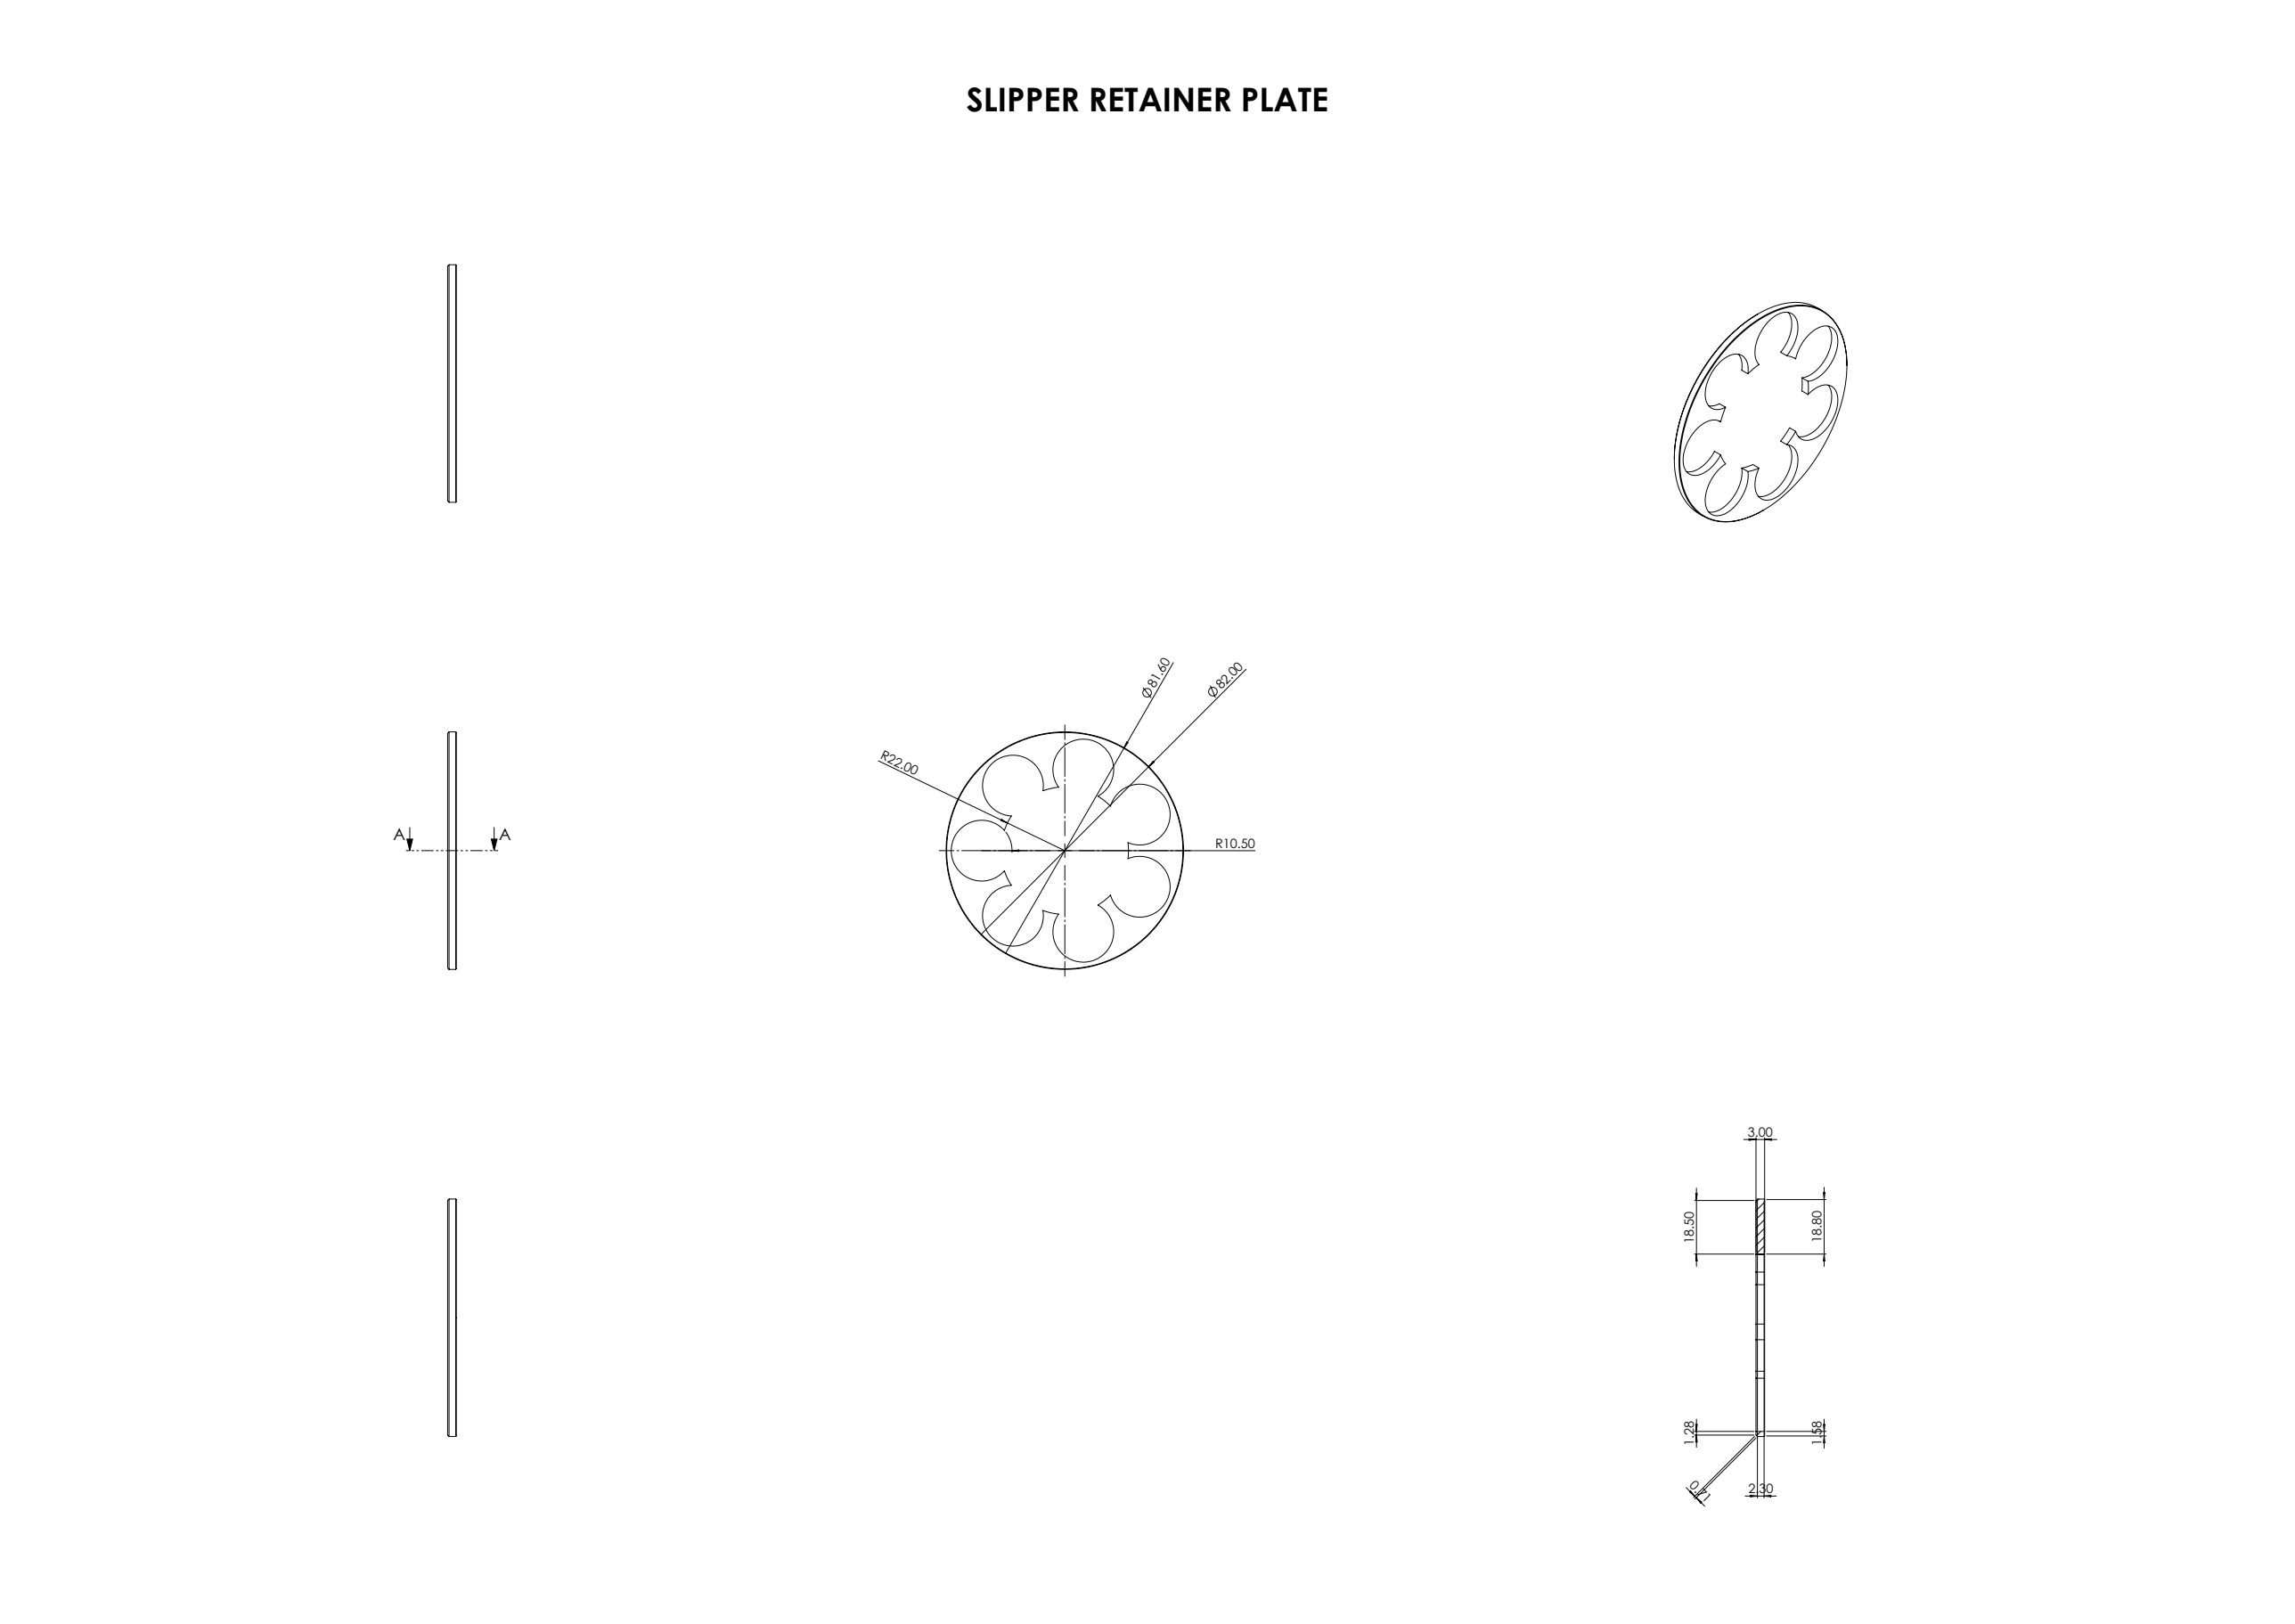
ISO-10303-21;
HEADER;
/* Generated by software containing ST-Developer
 * from STEP Tools, Inc. (www.steptools.com) 
 */

FILE_DESCRIPTION(
/* description */ (''),
/* implementation_level */ '2;1');

FILE_NAME(
/* name */ '07_Slipper_Retainer_Plate.step',
/* time_stamp */ '2026-10-26T07:49:00-07:00',
/* author */ (''),
/* organization */ (''),
/* preprocessor_version */ 'ST-DEVELOPER v20.2',
/* originating_system */ 'Autodesk Translation Framework v15.15.0.0',
/* authorisation */ '');

FILE_SCHEMA (('AUTOMOTIVE_DESIGN { 1 0 10303 214 3 1 1 }'));
ENDSEC;

DATA;
#10=MECHANICAL_DESIGN_GEOMETRIC_PRESENTATION_REPRESENTATION('',(#189),#38507);
#159=SHAPE_REPRESENTATION_RELATIONSHIP('SRR','None',#38587,#174);
#174=ADVANCED_BREP_SHAPE_REPRESENTATION('',(#204),#38504);
#189=STYLED_ITEM('',(#38713),#204);
#204=MANIFOLD_SOLID_BREP('Body1',#15083);
#515=FACE_BOUND('',#3178,.T.);
#516=FACE_BOUND('',#3194,.T.);
#809=PLANE('',#16309);
#810=PLANE('',#16352);
#1513=CYLINDRICAL_SURFACE('',#16324,41.);
#1514=CYLINDRICAL_SURFACE('',#16326,10.5);
#1515=CYLINDRICAL_SURFACE('',#16328,22.);
#1516=CYLINDRICAL_SURFACE('',#16330,10.5);
#1517=CYLINDRICAL_SURFACE('',#16332,22.);
#1518=CYLINDRICAL_SURFACE('',#16334,10.5);
#1519=CYLINDRICAL_SURFACE('',#16336,22.);
#1520=CYLINDRICAL_SURFACE('',#16338,10.5);
#1521=CYLINDRICAL_SURFACE('',#16340,22.);
#1522=CYLINDRICAL_SURFACE('',#16342,10.5);
#1523=CYLINDRICAL_SURFACE('',#16344,22.);
#1524=CYLINDRICAL_SURFACE('',#16346,10.5);
#1525=CYLINDRICAL_SURFACE('',#16348,22.);
#1526=CYLINDRICAL_SURFACE('',#16350,10.5);
#1527=CYLINDRICAL_SURFACE('',#16355,22.);
#2191=FACE_OUTER_BOUND('',#3176,.T.);
#2192=FACE_OUTER_BOUND('',#3177,.T.);
#2193=FACE_OUTER_BOUND('',#3179,.T.);
#2194=FACE_OUTER_BOUND('',#3180,.T.);
#2195=FACE_OUTER_BOUND('',#3181,.T.);
#2196=FACE_OUTER_BOUND('',#3182,.T.);
#2197=FACE_OUTER_BOUND('',#3183,.T.);
#2198=FACE_OUTER_BOUND('',#3184,.T.);
#2199=FACE_OUTER_BOUND('',#3185,.T.);
#2200=FACE_OUTER_BOUND('',#3186,.T.);
#2201=FACE_OUTER_BOUND('',#3187,.T.);
#2202=FACE_OUTER_BOUND('',#3188,.T.);
#2203=FACE_OUTER_BOUND('',#3189,.T.);
#2204=FACE_OUTER_BOUND('',#3190,.T.);
#2205=FACE_OUTER_BOUND('',#3191,.T.);
#2206=FACE_OUTER_BOUND('',#3192,.T.);
#2207=FACE_OUTER_BOUND('',#3193,.T.);
#2208=FACE_OUTER_BOUND('',#3195,.T.);
#2209=FACE_OUTER_BOUND('',#3196,.T.);
#3176=EDGE_LOOP('',(#12565,#12566,#12567,#12568,#12569));
#3177=EDGE_LOOP('',(#12570));
#3178=EDGE_LOOP('',(#12571,#12572,#12573,#12574,#12575,#12576,#12577,#12578,
#12579,#12580,#12581,#12582,#12583,#12584));
#3179=EDGE_LOOP('',(#12585,#12586,#12587,#12588,#12589));
#3180=EDGE_LOOP('',(#12590,#12591,#12592,#12593));
#3181=EDGE_LOOP('',(#12594,#12595,#12596,#12597));
#3182=EDGE_LOOP('',(#12598,#12599,#12600,#12601));
#3183=EDGE_LOOP('',(#12602,#12603,#12604,#12605));
#3184=EDGE_LOOP('',(#12606,#12607,#12608,#12609));
#3185=EDGE_LOOP('',(#12610,#12611,#12612,#12613));
#3186=EDGE_LOOP('',(#12614,#12615,#12616,#12617));
#3187=EDGE_LOOP('',(#12618,#12619,#12620,#12621));
#3188=EDGE_LOOP('',(#12622,#12623,#12624,#12625));
#3189=EDGE_LOOP('',(#12626,#12627,#12628,#12629));
#3190=EDGE_LOOP('',(#12630,#12631,#12632,#12633));
#3191=EDGE_LOOP('',(#12634,#12635,#12636,#12637));
#3192=EDGE_LOOP('',(#12638,#12639,#12640,#12641));
#3193=EDGE_LOOP('',(#12642));
#3194=EDGE_LOOP('',(#12643,#12644,#12645,#12646,#12647,#12648,#12649,#12650,
#12651,#12652,#12653,#12654,#12655,#12656));
#3195=EDGE_LOOP('',(#12657,#12658,#12659,#12660));
#3196=EDGE_LOOP('',(#12661,#12662,#12663,#12664));
#4141=LINE('',#27131,#5210);
#4142=LINE('',#27166,#5211);
#4143=LINE('',#27172,#5212);
#4144=LINE('',#27173,#5213);
#4145=LINE('',#27177,#5214);
#4146=LINE('',#27181,#5215);
#4147=LINE('',#27185,#5216);
#4148=LINE('',#27189,#5217);
#4149=LINE('',#27193,#5218);
#4150=LINE('',#27197,#5219);
#4151=LINE('',#27201,#5220);
#4152=LINE('',#27205,#5221);
#4153=LINE('',#27209,#5222);
#4154=LINE('',#27213,#5223);
#4155=LINE('',#27217,#5224);
#4156=LINE('',#27221,#5225);
#4157=LINE('',#27228,#5226);
#5210=VECTOR('',#19494,40.9);
#5211=VECTOR('',#19531,41.);
#5212=VECTOR('',#19538,10.);
#5213=VECTOR('',#19539,10.);
#5214=VECTOR('',#19544,10.);
#5215=VECTOR('',#19549,10.);
#5216=VECTOR('',#19554,10.);
#5217=VECTOR('',#19559,10.);
#5218=VECTOR('',#19564,10.);
#5219=VECTOR('',#19569,10.);
#5220=VECTOR('',#19574,10.);
#5221=VECTOR('',#19579,10.);
#5222=VECTOR('',#19584,10.);
#5223=VECTOR('',#19589,10.);
#5224=VECTOR('',#19594,10.);
#5225=VECTOR('',#19599,10.);
#5226=VECTOR('',#19610,40.75);
#6142=CIRCLE('',#16306,40.8);
#6143=CIRCLE('',#16307,41.);
#6144=CIRCLE('',#16308,41.);
#6145=CIRCLE('',#16310,10.5);
#6146=CIRCLE('',#16311,22.);
#6147=CIRCLE('',#16312,10.5);
#6148=CIRCLE('',#16313,22.);
#6149=CIRCLE('',#16314,10.5);
#6150=CIRCLE('',#16315,22.);
#6151=CIRCLE('',#16316,10.5);
#6152=CIRCLE('',#16317,22.);
#6153=CIRCLE('',#16318,10.5);
#6154=CIRCLE('',#16319,22.);
#6155=CIRCLE('',#16320,10.5);
#6156=CIRCLE('',#16321,22.);
#6157=CIRCLE('',#16322,10.5);
#6158=CIRCLE('',#16323,22.);
#6159=CIRCLE('',#16325,41.);
#6160=CIRCLE('',#16327,10.5);
#6161=CIRCLE('',#16329,22.);
#6162=CIRCLE('',#16331,10.5);
#6163=CIRCLE('',#16333,22.);
#6164=CIRCLE('',#16335,10.5);
#6165=CIRCLE('',#16337,22.);
#6166=CIRCLE('',#16339,10.5);
#6167=CIRCLE('',#16341,22.);
#6168=CIRCLE('',#16343,10.5);
#6169=CIRCLE('',#16345,22.);
#6170=CIRCLE('',#16347,10.5);
#6171=CIRCLE('',#16349,22.);
#6172=CIRCLE('',#16351,10.5);
#6173=CIRCLE('',#16353,40.5);
#6174=CIRCLE('',#16354,22.);
#7146=VERTEX_POINT('',#27128);
#7147=VERTEX_POINT('',#27130);
#7148=VERTEX_POINT('',#27132);
#7149=VERTEX_POINT('',#27136);
#7150=VERTEX_POINT('',#27137);
#7151=VERTEX_POINT('',#27139);
#7152=VERTEX_POINT('',#27141);
#7153=VERTEX_POINT('',#27143);
#7154=VERTEX_POINT('',#27145);
#7155=VERTEX_POINT('',#27147);
#7156=VERTEX_POINT('',#27149);
#7157=VERTEX_POINT('',#27151);
#7158=VERTEX_POINT('',#27153);
#7159=VERTEX_POINT('',#27155);
#7160=VERTEX_POINT('',#27157);
#7161=VERTEX_POINT('',#27159);
#7162=VERTEX_POINT('',#27161);
#7163=VERTEX_POINT('',#27165);
#7164=VERTEX_POINT('',#27169);
#7165=VERTEX_POINT('',#27170);
#7166=VERTEX_POINT('',#27175);
#7167=VERTEX_POINT('',#27179);
#7168=VERTEX_POINT('',#27183);
#7169=VERTEX_POINT('',#27187);
#7170=VERTEX_POINT('',#27191);
#7171=VERTEX_POINT('',#27195);
#7172=VERTEX_POINT('',#27199);
#7173=VERTEX_POINT('',#27203);
#7174=VERTEX_POINT('',#27207);
#7175=VERTEX_POINT('',#27211);
#7176=VERTEX_POINT('',#27215);
#7177=VERTEX_POINT('',#27219);
#7178=VERTEX_POINT('',#27223);
#9031=EDGE_CURVE('',#7146,#7146,#6142,.T.);
#9032=EDGE_CURVE('',#7146,#7147,#4141,.T.);
#9033=EDGE_CURVE('',#7147,#7148,#6143,.T.);
#9034=EDGE_CURVE('',#7148,#7147,#6144,.T.);
#9035=EDGE_CURVE('',#7149,#7150,#6145,.T.);
#9036=EDGE_CURVE('',#7151,#7150,#6146,.T.);
#9037=EDGE_CURVE('',#7151,#7152,#6147,.T.);
#9038=EDGE_CURVE('',#7153,#7152,#6148,.T.);
#9039=EDGE_CURVE('',#7153,#7154,#6149,.T.);
#9040=EDGE_CURVE('',#7155,#7154,#6150,.T.);
#9041=EDGE_CURVE('',#7155,#7156,#6151,.T.);
#9042=EDGE_CURVE('',#7157,#7156,#6152,.T.);
#9043=EDGE_CURVE('',#7157,#7158,#6153,.T.);
#9044=EDGE_CURVE('',#7159,#7158,#6154,.T.);
#9045=EDGE_CURVE('',#7159,#7160,#6155,.T.);
#9046=EDGE_CURVE('',#7161,#7160,#6156,.T.);
#9047=EDGE_CURVE('',#7161,#7162,#6157,.T.);
#9048=EDGE_CURVE('',#7149,#7162,#6158,.T.);
#9049=EDGE_CURVE('',#7148,#7163,#4142,.T.);
#9050=EDGE_CURVE('',#7163,#7163,#6159,.T.);
#9051=EDGE_CURVE('',#7164,#7165,#6160,.T.);
#9052=EDGE_CURVE('',#7150,#7164,#4143,.T.);
#9053=EDGE_CURVE('',#7165,#7149,#4144,.T.);
#9054=EDGE_CURVE('',#7166,#7164,#6161,.T.);
#9055=EDGE_CURVE('',#7166,#7151,#4145,.T.);
#9056=EDGE_CURVE('',#7167,#7166,#6162,.T.);
#9057=EDGE_CURVE('',#7152,#7167,#4146,.T.);
#9058=EDGE_CURVE('',#7168,#7167,#6163,.T.);
#9059=EDGE_CURVE('',#7168,#7153,#4147,.T.);
#9060=EDGE_CURVE('',#7169,#7168,#6164,.T.);
#9061=EDGE_CURVE('',#7154,#7169,#4148,.T.);
#9062=EDGE_CURVE('',#7170,#7169,#6165,.T.);
#9063=EDGE_CURVE('',#7170,#7155,#4149,.T.);
#9064=EDGE_CURVE('',#7171,#7170,#6166,.T.);
#9065=EDGE_CURVE('',#7156,#7171,#4150,.T.);
#9066=EDGE_CURVE('',#7172,#7171,#6167,.T.);
#9067=EDGE_CURVE('',#7172,#7157,#4151,.T.);
#9068=EDGE_CURVE('',#7173,#7172,#6168,.T.);
#9069=EDGE_CURVE('',#7158,#7173,#4152,.T.);
#9070=EDGE_CURVE('',#7174,#7173,#6169,.T.);
#9071=EDGE_CURVE('',#7174,#7159,#4153,.T.);
#9072=EDGE_CURVE('',#7175,#7174,#6170,.T.);
#9073=EDGE_CURVE('',#7160,#7175,#4154,.T.);
#9074=EDGE_CURVE('',#7176,#7175,#6171,.T.);
#9075=EDGE_CURVE('',#7176,#7161,#4155,.T.);
#9076=EDGE_CURVE('',#7177,#7176,#6172,.T.);
#9077=EDGE_CURVE('',#7162,#7177,#4156,.T.);
#9078=EDGE_CURVE('',#7178,#7178,#6173,.T.);
#9079=EDGE_CURVE('',#7165,#7177,#6174,.T.);
#9080=EDGE_CURVE('',#7163,#7178,#4157,.T.);
#12565=ORIENTED_EDGE('',*,*,#9031,.T.);
#12566=ORIENTED_EDGE('',*,*,#9032,.T.);
#12567=ORIENTED_EDGE('',*,*,#9033,.T.);
#12568=ORIENTED_EDGE('',*,*,#9034,.T.);
#12569=ORIENTED_EDGE('',*,*,#9032,.F.);
#12570=ORIENTED_EDGE('',*,*,#9031,.F.);
#12571=ORIENTED_EDGE('',*,*,#9035,.T.);
#12572=ORIENTED_EDGE('',*,*,#9036,.F.);
#12573=ORIENTED_EDGE('',*,*,#9037,.T.);
#12574=ORIENTED_EDGE('',*,*,#9038,.F.);
#12575=ORIENTED_EDGE('',*,*,#9039,.T.);
#12576=ORIENTED_EDGE('',*,*,#9040,.F.);
#12577=ORIENTED_EDGE('',*,*,#9041,.T.);
#12578=ORIENTED_EDGE('',*,*,#9042,.F.);
#12579=ORIENTED_EDGE('',*,*,#9043,.T.);
#12580=ORIENTED_EDGE('',*,*,#9044,.F.);
#12581=ORIENTED_EDGE('',*,*,#9045,.T.);
#12582=ORIENTED_EDGE('',*,*,#9046,.F.);
#12583=ORIENTED_EDGE('',*,*,#9047,.T.);
#12584=ORIENTED_EDGE('',*,*,#9048,.F.);
#12585=ORIENTED_EDGE('',*,*,#9033,.F.);
#12586=ORIENTED_EDGE('',*,*,#9034,.F.);
#12587=ORIENTED_EDGE('',*,*,#9049,.T.);
#12588=ORIENTED_EDGE('',*,*,#9050,.T.);
#12589=ORIENTED_EDGE('',*,*,#9049,.F.);
#12590=ORIENTED_EDGE('',*,*,#9051,.F.);
#12591=ORIENTED_EDGE('',*,*,#9052,.F.);
#12592=ORIENTED_EDGE('',*,*,#9035,.F.);
#12593=ORIENTED_EDGE('',*,*,#9053,.F.);
#12594=ORIENTED_EDGE('',*,*,#9052,.T.);
#12595=ORIENTED_EDGE('',*,*,#9054,.F.);
#12596=ORIENTED_EDGE('',*,*,#9055,.T.);
#12597=ORIENTED_EDGE('',*,*,#9036,.T.);
#12598=ORIENTED_EDGE('',*,*,#9056,.F.);
#12599=ORIENTED_EDGE('',*,*,#9057,.F.);
#12600=ORIENTED_EDGE('',*,*,#9037,.F.);
#12601=ORIENTED_EDGE('',*,*,#9055,.F.);
#12602=ORIENTED_EDGE('',*,*,#9057,.T.);
#12603=ORIENTED_EDGE('',*,*,#9058,.F.);
#12604=ORIENTED_EDGE('',*,*,#9059,.T.);
#12605=ORIENTED_EDGE('',*,*,#9038,.T.);
#12606=ORIENTED_EDGE('',*,*,#9060,.F.);
#12607=ORIENTED_EDGE('',*,*,#9061,.F.);
#12608=ORIENTED_EDGE('',*,*,#9039,.F.);
#12609=ORIENTED_EDGE('',*,*,#9059,.F.);
#12610=ORIENTED_EDGE('',*,*,#9061,.T.);
#12611=ORIENTED_EDGE('',*,*,#9062,.F.);
#12612=ORIENTED_EDGE('',*,*,#9063,.T.);
#12613=ORIENTED_EDGE('',*,*,#9040,.T.);
#12614=ORIENTED_EDGE('',*,*,#9064,.F.);
#12615=ORIENTED_EDGE('',*,*,#9065,.F.);
#12616=ORIENTED_EDGE('',*,*,#9041,.F.);
#12617=ORIENTED_EDGE('',*,*,#9063,.F.);
#12618=ORIENTED_EDGE('',*,*,#9065,.T.);
#12619=ORIENTED_EDGE('',*,*,#9066,.F.);
#12620=ORIENTED_EDGE('',*,*,#9067,.T.);
#12621=ORIENTED_EDGE('',*,*,#9042,.T.);
#12622=ORIENTED_EDGE('',*,*,#9068,.F.);
#12623=ORIENTED_EDGE('',*,*,#9069,.F.);
#12624=ORIENTED_EDGE('',*,*,#9043,.F.);
#12625=ORIENTED_EDGE('',*,*,#9067,.F.);
#12626=ORIENTED_EDGE('',*,*,#9069,.T.);
#12627=ORIENTED_EDGE('',*,*,#9070,.F.);
#12628=ORIENTED_EDGE('',*,*,#9071,.T.);
#12629=ORIENTED_EDGE('',*,*,#9044,.T.);
#12630=ORIENTED_EDGE('',*,*,#9072,.F.);
#12631=ORIENTED_EDGE('',*,*,#9073,.F.);
#12632=ORIENTED_EDGE('',*,*,#9045,.F.);
#12633=ORIENTED_EDGE('',*,*,#9071,.F.);
#12634=ORIENTED_EDGE('',*,*,#9073,.T.);
#12635=ORIENTED_EDGE('',*,*,#9074,.F.);
#12636=ORIENTED_EDGE('',*,*,#9075,.T.);
#12637=ORIENTED_EDGE('',*,*,#9046,.T.);
#12638=ORIENTED_EDGE('',*,*,#9075,.F.);
#12639=ORIENTED_EDGE('',*,*,#9076,.F.);
#12640=ORIENTED_EDGE('',*,*,#9077,.F.);
#12641=ORIENTED_EDGE('',*,*,#9047,.F.);
#12642=ORIENTED_EDGE('',*,*,#9078,.F.);
#12643=ORIENTED_EDGE('',*,*,#9051,.T.);
#12644=ORIENTED_EDGE('',*,*,#9079,.T.);
#12645=ORIENTED_EDGE('',*,*,#9076,.T.);
#12646=ORIENTED_EDGE('',*,*,#9074,.T.);
#12647=ORIENTED_EDGE('',*,*,#9072,.T.);
#12648=ORIENTED_EDGE('',*,*,#9070,.T.);
#12649=ORIENTED_EDGE('',*,*,#9068,.T.);
#12650=ORIENTED_EDGE('',*,*,#9066,.T.);
#12651=ORIENTED_EDGE('',*,*,#9064,.T.);
#12652=ORIENTED_EDGE('',*,*,#9062,.T.);
#12653=ORIENTED_EDGE('',*,*,#9060,.T.);
#12654=ORIENTED_EDGE('',*,*,#9058,.T.);
#12655=ORIENTED_EDGE('',*,*,#9056,.T.);
#12656=ORIENTED_EDGE('',*,*,#9054,.T.);
#12657=ORIENTED_EDGE('',*,*,#9053,.T.);
#12658=ORIENTED_EDGE('',*,*,#9048,.T.);
#12659=ORIENTED_EDGE('',*,*,#9077,.T.);
#12660=ORIENTED_EDGE('',*,*,#9079,.F.);
#12661=ORIENTED_EDGE('',*,*,#9050,.F.);
#12662=ORIENTED_EDGE('',*,*,#9080,.T.);
#12663=ORIENTED_EDGE('',*,*,#9078,.T.);
#12664=ORIENTED_EDGE('',*,*,#9080,.F.);
#14179=CONICAL_SURFACE('',#16305,40.9,0.785398163397437);
#14180=CONICAL_SURFACE('',#16356,40.75,0.785398163397447);
#14758=ADVANCED_FACE('',(#2191),#14179,.T.);
#14759=ADVANCED_FACE('',(#2192,#515),#809,.T.);
#14760=ADVANCED_FACE('',(#2193),#1513,.T.);
#14761=ADVANCED_FACE('',(#2194),#1514,.F.);
#14762=ADVANCED_FACE('',(#2195),#1515,.F.);
#14763=ADVANCED_FACE('',(#2196),#1516,.F.);
#14764=ADVANCED_FACE('',(#2197),#1517,.F.);
#14765=ADVANCED_FACE('',(#2198),#1518,.F.);
#14766=ADVANCED_FACE('',(#2199),#1519,.F.);
#14767=ADVANCED_FACE('',(#2200),#1520,.F.);
#14768=ADVANCED_FACE('',(#2201),#1521,.F.);
#14769=ADVANCED_FACE('',(#2202),#1522,.F.);
#14770=ADVANCED_FACE('',(#2203),#1523,.F.);
#14771=ADVANCED_FACE('',(#2204),#1524,.F.);
#14772=ADVANCED_FACE('',(#2205),#1525,.F.);
#14773=ADVANCED_FACE('',(#2206),#1526,.F.);
#14774=ADVANCED_FACE('',(#2207,#516),#810,.T.);
#14775=ADVANCED_FACE('',(#2208),#1527,.F.);
#14776=ADVANCED_FACE('',(#2209),#14180,.T.);
#15083=CLOSED_SHELL('',(#14758,#14759,#14760,#14761,#14762,#14763,#14764,
#14765,#14766,#14767,#14768,#14769,#14770,#14771,#14772,#14773,#14774,#14775,
#14776));
#16304=AXIS2_PLACEMENT_3D('',#27126,#19488,#19489);
#16305=AXIS2_PLACEMENT_3D('',#27127,#19490,#19491);
#16306=AXIS2_PLACEMENT_3D('',#27129,#19492,#19493);
#16307=AXIS2_PLACEMENT_3D('',#27133,#19495,#19496);
#16308=AXIS2_PLACEMENT_3D('',#27134,#19497,#19498);
#16309=AXIS2_PLACEMENT_3D('',#27135,#19499,#19500);
#16310=AXIS2_PLACEMENT_3D('',#27138,#19501,#19502);
#16311=AXIS2_PLACEMENT_3D('',#27140,#19503,#19504);
#16312=AXIS2_PLACEMENT_3D('',#27142,#19505,#19506);
#16313=AXIS2_PLACEMENT_3D('',#27144,#19507,#19508);
#16314=AXIS2_PLACEMENT_3D('',#27146,#19509,#19510);
#16315=AXIS2_PLACEMENT_3D('',#27148,#19511,#19512);
#16316=AXIS2_PLACEMENT_3D('',#27150,#19513,#19514);
#16317=AXIS2_PLACEMENT_3D('',#27152,#19515,#19516);
#16318=AXIS2_PLACEMENT_3D('',#27154,#19517,#19518);
#16319=AXIS2_PLACEMENT_3D('',#27156,#19519,#19520);
#16320=AXIS2_PLACEMENT_3D('',#27158,#19521,#19522);
#16321=AXIS2_PLACEMENT_3D('',#27160,#19523,#19524);
#16322=AXIS2_PLACEMENT_3D('',#27162,#19525,#19526);
#16323=AXIS2_PLACEMENT_3D('',#27163,#19527,#19528);
#16324=AXIS2_PLACEMENT_3D('',#27164,#19529,#19530);
#16325=AXIS2_PLACEMENT_3D('',#27167,#19532,#19533);
#16326=AXIS2_PLACEMENT_3D('',#27168,#19534,#19535);
#16327=AXIS2_PLACEMENT_3D('',#27171,#19536,#19537);
#16328=AXIS2_PLACEMENT_3D('',#27174,#19540,#19541);
#16329=AXIS2_PLACEMENT_3D('',#27176,#19542,#19543);
#16330=AXIS2_PLACEMENT_3D('',#27178,#19545,#19546);
#16331=AXIS2_PLACEMENT_3D('',#27180,#19547,#19548);
#16332=AXIS2_PLACEMENT_3D('',#27182,#19550,#19551);
#16333=AXIS2_PLACEMENT_3D('',#27184,#19552,#19553);
#16334=AXIS2_PLACEMENT_3D('',#27186,#19555,#19556);
#16335=AXIS2_PLACEMENT_3D('',#27188,#19557,#19558);
#16336=AXIS2_PLACEMENT_3D('',#27190,#19560,#19561);
#16337=AXIS2_PLACEMENT_3D('',#27192,#19562,#19563);
#16338=AXIS2_PLACEMENT_3D('',#27194,#19565,#19566);
#16339=AXIS2_PLACEMENT_3D('',#27196,#19567,#19568);
#16340=AXIS2_PLACEMENT_3D('',#27198,#19570,#19571);
#16341=AXIS2_PLACEMENT_3D('',#27200,#19572,#19573);
#16342=AXIS2_PLACEMENT_3D('',#27202,#19575,#19576);
#16343=AXIS2_PLACEMENT_3D('',#27204,#19577,#19578);
#16344=AXIS2_PLACEMENT_3D('',#27206,#19580,#19581);
#16345=AXIS2_PLACEMENT_3D('',#27208,#19582,#19583);
#16346=AXIS2_PLACEMENT_3D('',#27210,#19585,#19586);
#16347=AXIS2_PLACEMENT_3D('',#27212,#19587,#19588);
#16348=AXIS2_PLACEMENT_3D('',#27214,#19590,#19591);
#16349=AXIS2_PLACEMENT_3D('',#27216,#19592,#19593);
#16350=AXIS2_PLACEMENT_3D('',#27218,#19595,#19596);
#16351=AXIS2_PLACEMENT_3D('',#27220,#19597,#19598);
#16352=AXIS2_PLACEMENT_3D('',#27222,#19600,#19601);
#16353=AXIS2_PLACEMENT_3D('',#27224,#19602,#19603);
#16354=AXIS2_PLACEMENT_3D('',#27225,#19604,#19605);
#16355=AXIS2_PLACEMENT_3D('',#27226,#19606,#19607);
#16356=AXIS2_PLACEMENT_3D('',#27227,#19608,#19609);
#19488=DIRECTION('axis',(0.,0.,1.));
#19489=DIRECTION('refdir',(1.,0.,0.));
#19490=DIRECTION('center_axis',(-1.,0.,0.));
#19491=DIRECTION('ref_axis',(0.,-1.,0.));
#19492=DIRECTION('center_axis',(-1.,0.,0.));
#19493=DIRECTION('ref_axis',(0.,-1.,0.));
#19494=DIRECTION('',(-0.707106781186555,0.70710678118654,8.65956056235484E-17));
#19495=DIRECTION('center_axis',(1.,0.,0.));
#19496=DIRECTION('ref_axis',(0.,-1.,0.));
#19497=DIRECTION('center_axis',(1.,0.,0.));
#19498=DIRECTION('ref_axis',(0.,-1.,0.));
#19499=DIRECTION('center_axis',(1.,0.,0.));
#19500=DIRECTION('ref_axis',(0.,0.,-1.));
#19501=DIRECTION('center_axis',(-1.,0.,0.));
#19502=DIRECTION('ref_axis',(0.,-0.78183148246803,-0.623489801858733));
#19503=DIRECTION('center_axis',(1.,0.,0.));
#19504=DIRECTION('ref_axis',(0.,0.,-1.));
#19505=DIRECTION('center_axis',(-1.,0.,0.));
#19506=DIRECTION('ref_axis',(0.,-0.974927912181824,0.222520933956315));
#19507=DIRECTION('center_axis',(1.,0.,0.));
#19508=DIRECTION('ref_axis',(0.,0.,-1.));
#19509=DIRECTION('center_axis',(-1.,0.,0.));
#19510=DIRECTION('ref_axis',(0.,-0.433883739117558,0.900968867902419));
#19511=DIRECTION('center_axis',(1.,0.,0.));
#19512=DIRECTION('ref_axis',(0.,0.,-1.));
#19513=DIRECTION('center_axis',(-1.,0.,0.));
#19514=DIRECTION('ref_axis',(0.,0.433883739117558,0.900968867902419));
#19515=DIRECTION('center_axis',(1.,0.,0.));
#19516=DIRECTION('ref_axis',(0.,0.,-1.));
#19517=DIRECTION('center_axis',(-1.,0.,0.));
#19518=DIRECTION('ref_axis',(0.,0.974927912181824,0.222520933956314));
#19519=DIRECTION('center_axis',(1.,0.,0.));
#19520=DIRECTION('ref_axis',(0.,0.,-1.));
#19521=DIRECTION('center_axis',(-1.,0.,0.));
#19522=DIRECTION('ref_axis',(0.,0.78183148246803,-0.623489801858734));
#19523=DIRECTION('center_axis',(1.,0.,0.));
#19524=DIRECTION('ref_axis',(0.,0.,-1.));
#19525=DIRECTION('center_axis',(-1.,0.,0.));
#19526=DIRECTION('ref_axis',(0.,0.,-1.));
#19527=DIRECTION('center_axis',(1.,0.,0.));
#19528=DIRECTION('ref_axis',(0.,0.,-1.));
#19529=DIRECTION('center_axis',(1.,0.,0.));
#19530=DIRECTION('ref_axis',(0.,1.,0.));
#19531=DIRECTION('',(-1.,0.,0.));
#19532=DIRECTION('center_axis',(1.,0.,0.));
#19533=DIRECTION('ref_axis',(0.,0.,-1.));
#19534=DIRECTION('center_axis',(1.,0.,0.));
#19535=DIRECTION('ref_axis',(0.,0.78183148246803,0.623489801858733));
#19536=DIRECTION('center_axis',(1.,0.,0.));
#19537=DIRECTION('ref_axis',(0.,-0.78183148246803,-0.623489801858733));
#19538=DIRECTION('',(-1.,0.,0.));
#19539=DIRECTION('',(1.,0.,0.));
#19540=DIRECTION('center_axis',(1.,0.,0.));
#19541=DIRECTION('ref_axis',(0.,1.,0.));
#19542=DIRECTION('center_axis',(1.,0.,0.));
#19543=DIRECTION('ref_axis',(0.,0.,-1.));
#19544=DIRECTION('',(1.,0.,0.));
#19545=DIRECTION('center_axis',(1.,0.,0.));
#19546=DIRECTION('ref_axis',(0.,0.974927912181824,-0.222520933956315));
#19547=DIRECTION('center_axis',(1.,0.,0.));
#19548=DIRECTION('ref_axis',(0.,-0.974927912181824,0.222520933956315));
#19549=DIRECTION('',(-1.,0.,0.));
#19550=DIRECTION('center_axis',(1.,0.,0.));
#19551=DIRECTION('ref_axis',(0.,1.,0.));
#19552=DIRECTION('center_axis',(1.,0.,0.));
#19553=DIRECTION('ref_axis',(0.,0.,-1.));
#19554=DIRECTION('',(1.,0.,0.));
#19555=DIRECTION('center_axis',(1.,0.,0.));
#19556=DIRECTION('ref_axis',(0.,0.433883739117558,-0.900968867902419));
#19557=DIRECTION('center_axis',(1.,0.,0.));
#19558=DIRECTION('ref_axis',(0.,-0.433883739117558,0.900968867902419));
#19559=DIRECTION('',(-1.,0.,0.));
#19560=DIRECTION('center_axis',(1.,0.,0.));
#19561=DIRECTION('ref_axis',(0.,1.,0.));
#19562=DIRECTION('center_axis',(1.,0.,0.));
#19563=DIRECTION('ref_axis',(0.,0.,-1.));
#19564=DIRECTION('',(1.,0.,0.));
#19565=DIRECTION('center_axis',(1.,0.,0.));
#19566=DIRECTION('ref_axis',(0.,-0.433883739117558,-0.900968867902419));
#19567=DIRECTION('center_axis',(1.,0.,0.));
#19568=DIRECTION('ref_axis',(0.,0.433883739117558,0.900968867902419));
#19569=DIRECTION('',(-1.,0.,0.));
#19570=DIRECTION('center_axis',(1.,0.,0.));
#19571=DIRECTION('ref_axis',(0.,1.,0.));
#19572=DIRECTION('center_axis',(1.,0.,0.));
#19573=DIRECTION('ref_axis',(0.,0.,-1.));
#19574=DIRECTION('',(1.,0.,0.));
#19575=DIRECTION('center_axis',(1.,0.,0.));
#19576=DIRECTION('ref_axis',(0.,-0.974927912181824,-0.222520933956314));
#19577=DIRECTION('center_axis',(1.,0.,0.));
#19578=DIRECTION('ref_axis',(0.,0.974927912181824,0.222520933956314));
#19579=DIRECTION('',(-1.,0.,0.));
#19580=DIRECTION('center_axis',(1.,0.,0.));
#19581=DIRECTION('ref_axis',(0.,1.,0.));
#19582=DIRECTION('center_axis',(1.,0.,0.));
#19583=DIRECTION('ref_axis',(0.,0.,-1.));
#19584=DIRECTION('',(1.,0.,0.));
#19585=DIRECTION('center_axis',(1.,0.,0.));
#19586=DIRECTION('ref_axis',(0.,-0.78183148246803,0.623489801858734));
#19587=DIRECTION('center_axis',(1.,0.,0.));
#19588=DIRECTION('ref_axis',(0.,0.78183148246803,-0.623489801858734));
#19589=DIRECTION('',(-1.,0.,0.));
#19590=DIRECTION('center_axis',(1.,0.,0.));
#19591=DIRECTION('ref_axis',(0.,1.,0.));
#19592=DIRECTION('center_axis',(1.,0.,0.));
#19593=DIRECTION('ref_axis',(0.,0.,-1.));
#19594=DIRECTION('',(1.,0.,0.));
#19595=DIRECTION('center_axis',(1.,0.,0.));
#19596=DIRECTION('ref_axis',(0.,-1.22464679914735E-16,1.));
#19597=DIRECTION('center_axis',(1.,0.,0.));
#19598=DIRECTION('ref_axis',(0.,0.,-1.));
#19599=DIRECTION('',(-1.,0.,0.));
#19600=DIRECTION('center_axis',(-1.,0.,0.));
#19601=DIRECTION('ref_axis',(0.,0.,1.));
#19602=DIRECTION('center_axis',(1.,0.,0.));
#19603=DIRECTION('ref_axis',(0.,0.,-1.));
#19604=DIRECTION('center_axis',(1.,0.,0.));
#19605=DIRECTION('ref_axis',(0.,0.,-1.));
#19606=DIRECTION('center_axis',(1.,0.,0.));
#19607=DIRECTION('ref_axis',(0.,1.,0.));
#19608=DIRECTION('center_axis',(1.,0.,0.));
#19609=DIRECTION('ref_axis',(0.,1.,0.));
#19610=DIRECTION('',(-0.707106781186549,0.707106781186546,8.65956056235492E-17));
#27126=CARTESIAN_POINT('',(0.,0.,0.));
#27127=CARTESIAN_POINT('Origin',(6.9,0.,0.));
#27128=CARTESIAN_POINT('',(7.,40.8,-4.9965589405212E-15));
#27129=CARTESIAN_POINT('Origin',(7.,0.,0.));
#27130=CARTESIAN_POINT('',(6.8,41.,5.02105187650415E-15));
#27131=CARTESIAN_POINT('',(6.9,40.9,5.00880540851267E-15));
#27132=CARTESIAN_POINT('',(6.8,-41.,-5.02105187650415E-15));
#27133=CARTESIAN_POINT('Origin',(6.8,0.,0.));
#27134=CARTESIAN_POINT('Origin',(6.8,0.,0.));
#27135=CARTESIAN_POINT('Origin',(7.,22.,0.));
#27136=CARTESIAN_POINT('',(7.,11.9691009237861,18.4591609526604));
#27137=CARTESIAN_POINT('',(7.,20.6597267643837,7.56146083908438));
#27138=CARTESIAN_POINT('Origin',(7.,22.4545685280471,17.9069208599539));
#27139=CARTESIAN_POINT('',(7.,21.894565536133,2.15127868579955));
#27140=CARTESIAN_POINT('Origin',(7.,0.,0.));
#27141=CARTESIAN_POINT('',(7.,18.7929170842265,-11.4379310832593));
#27142=CARTESIAN_POINT('Origin',(7.,28.0003889647509,-6.39090606159037));
#27143=CARTESIAN_POINT('',(7.,15.3329757320272,-15.7765603095562));
#27144=CARTESIAN_POINT('Origin',(7.,0.,0.));
#27145=CARTESIAN_POINT('',(7.,2.77465753400022,-21.8243276086347));
#27146=CARTESIAN_POINT('Origin',(7.,12.4613454071529,-25.8762503680314));
#27147=CARTESIAN_POINT('',(7.,-2.77465753400023,-21.8243276086347));
#27148=CARTESIAN_POINT('Origin',(7.,0.,0.));
#27149=CARTESIAN_POINT('',(7.,-15.3329757320272,-15.7765603095562));
#27150=CARTESIAN_POINT('Origin',(7.,-12.4613454071529,-25.8762503680314));
#27151=CARTESIAN_POINT('',(7.,-18.7929170842265,-11.4379310832593));
#27152=CARTESIAN_POINT('Origin',(7.,0.,0.));
#27153=CARTESIAN_POINT('',(7.,-21.894565536133,2.15127868579957));
#27154=CARTESIAN_POINT('Origin',(7.,-28.0003889647509,-6.39090606159036));
#27155=CARTESIAN_POINT('',(7.,-20.6597267643837,7.56146083908439));
#27156=CARTESIAN_POINT('Origin',(7.,0.,0.));
#27157=CARTESIAN_POINT('',(7.,-11.9691009237861,18.4591609526604));
#27158=CARTESIAN_POINT('Origin',(7.,-22.4545685280471,17.9069208599539));
#27159=CARTESIAN_POINT('',(7.,-6.96934080933589,20.8669185239059));
#27160=CARTESIAN_POINT('Origin',(7.,0.,0.));
#27161=CARTESIAN_POINT('',(7.,6.96934080933589,20.8669185239059));
#27162=CARTESIAN_POINT('Origin',(7.,0.,28.7204711393357));
#27163=CARTESIAN_POINT('Origin',(7.,0.,0.));
#27164=CARTESIAN_POINT('Origin',(5.75,0.,0.));
#27165=CARTESIAN_POINT('',(4.5,-41.,-5.02105187650415E-15));
#27166=CARTESIAN_POINT('',(5.75,-41.,-5.02105187650415E-15));
#27167=CARTESIAN_POINT('Origin',(4.5,0.,0.));
#27168=CARTESIAN_POINT('Origin',(3.9,22.4545685280471,17.9069208599539));
#27169=CARTESIAN_POINT('',(4.,20.6597267643837,7.56146083908438));
#27170=CARTESIAN_POINT('',(4.,11.9691009237861,18.4591609526604));
#27171=CARTESIAN_POINT('Origin',(4.,22.4545685280471,17.9069208599539));
#27172=CARTESIAN_POINT('',(3.9,20.6597267643837,7.56146083908438));
#27173=CARTESIAN_POINT('',(3.9,11.9691009237861,18.4591609526604));
#27174=CARTESIAN_POINT('Origin',(5.5,0.,0.));
#27175=CARTESIAN_POINT('',(4.,21.894565536133,2.15127868579955));
#27176=CARTESIAN_POINT('Origin',(4.,0.,0.));
#27177=CARTESIAN_POINT('',(3.9,21.894565536133,2.15127868579956));
#27178=CARTESIAN_POINT('Origin',(3.9,28.0003889647509,-6.39090606159037));
#27179=CARTESIAN_POINT('',(4.,18.7929170842265,-11.4379310832593));
#27180=CARTESIAN_POINT('Origin',(4.,28.0003889647509,-6.39090606159037));
#27181=CARTESIAN_POINT('',(3.9,18.7929170842265,-11.4379310832593));
#27182=CARTESIAN_POINT('Origin',(5.5,0.,0.));
#27183=CARTESIAN_POINT('',(4.,15.3329757320272,-15.7765603095562));
#27184=CARTESIAN_POINT('Origin',(4.,0.,0.));
#27185=CARTESIAN_POINT('',(3.9,15.3329757320272,-15.7765603095562));
#27186=CARTESIAN_POINT('Origin',(3.9,12.4613454071529,-25.8762503680314));
#27187=CARTESIAN_POINT('',(4.,2.77465753400022,-21.8243276086347));
#27188=CARTESIAN_POINT('Origin',(4.,12.4613454071529,-25.8762503680314));
#27189=CARTESIAN_POINT('',(3.9,2.77465753400023,-21.8243276086347));
#27190=CARTESIAN_POINT('Origin',(5.5,0.,0.));
#27191=CARTESIAN_POINT('',(4.,-2.77465753400023,-21.8243276086347));
#27192=CARTESIAN_POINT('Origin',(4.,0.,0.));
#27193=CARTESIAN_POINT('',(3.9,-2.77465753400023,-21.8243276086347));
#27194=CARTESIAN_POINT('Origin',(3.9,-12.4613454071529,-25.8762503680314));
#27195=CARTESIAN_POINT('',(4.,-15.3329757320272,-15.7765603095562));
#27196=CARTESIAN_POINT('Origin',(4.,-12.4613454071529,-25.8762503680314));
#27197=CARTESIAN_POINT('',(3.9,-15.3329757320272,-15.7765603095562));
#27198=CARTESIAN_POINT('Origin',(5.5,0.,0.));
#27199=CARTESIAN_POINT('',(4.,-18.7929170842265,-11.4379310832593));
#27200=CARTESIAN_POINT('Origin',(4.,0.,0.));
#27201=CARTESIAN_POINT('',(3.9,-18.7929170842265,-11.4379310832593));
#27202=CARTESIAN_POINT('Origin',(3.9,-28.0003889647509,-6.39090606159036));
#27203=CARTESIAN_POINT('',(4.,-21.894565536133,2.15127868579957));
#27204=CARTESIAN_POINT('Origin',(4.,-28.0003889647509,-6.39090606159036));
#27205=CARTESIAN_POINT('',(3.9,-21.894565536133,2.15127868579957));
#27206=CARTESIAN_POINT('Origin',(5.5,0.,0.));
#27207=CARTESIAN_POINT('',(4.,-20.6597267643837,7.56146083908439));
#27208=CARTESIAN_POINT('Origin',(4.,0.,0.));
#27209=CARTESIAN_POINT('',(3.9,-20.6597267643837,7.56146083908439));
#27210=CARTESIAN_POINT('Origin',(3.9,-22.4545685280471,17.9069208599539));
#27211=CARTESIAN_POINT('',(4.,-11.9691009237861,18.4591609526604));
#27212=CARTESIAN_POINT('Origin',(4.,-22.4545685280471,17.9069208599539));
#27213=CARTESIAN_POINT('',(3.9,-11.9691009237861,18.4591609526604));
#27214=CARTESIAN_POINT('Origin',(5.5,0.,0.));
#27215=CARTESIAN_POINT('',(4.,-6.96934080933589,20.8669185239059));
#27216=CARTESIAN_POINT('Origin',(4.,0.,0.));
#27217=CARTESIAN_POINT('',(3.9,-6.96934080933589,20.8669185239059));
#27218=CARTESIAN_POINT('Origin',(3.9,0.,28.7204711393357));
#27219=CARTESIAN_POINT('',(4.,6.96934080933589,20.8669185239059));
#27220=CARTESIAN_POINT('Origin',(4.,0.,28.7204711393357));
#27221=CARTESIAN_POINT('',(3.9,6.96934080933589,20.8669185239059));
#27222=CARTESIAN_POINT('Origin',(4.,40.5,0.));
#27223=CARTESIAN_POINT('',(4.,-40.5,-4.95981953654678E-15));
#27224=CARTESIAN_POINT('Origin',(4.,0.,0.));
#27225=CARTESIAN_POINT('Origin',(4.,0.,0.));
#27226=CARTESIAN_POINT('Origin',(5.5,0.,0.));
#27227=CARTESIAN_POINT('Origin',(4.25,0.,0.));
#27228=CARTESIAN_POINT('',(4.25,-40.75,-4.99043570652546E-15));
#38487=UNCERTAINTY_MEASURE_WITH_UNIT(LENGTH_MEASURE(0.01),#38508,
'DISTANCE_ACCURACY_VALUE',
'Maximum model space distance between geometric entities at asserted c
onnectivities');
#38490=UNCERTAINTY_MEASURE_WITH_UNIT(LENGTH_MEASURE(0.01),#38508,
'DISTANCE_ACCURACY_VALUE',
'Maximum model space distance between geometric entities at asserted c
onnectivities');
#38504=(
GEOMETRIC_REPRESENTATION_CONTEXT(3)
GLOBAL_UNCERTAINTY_ASSIGNED_CONTEXT((#38487))
GLOBAL_UNIT_ASSIGNED_CONTEXT((#38508,#38510,#38511))
REPRESENTATION_CONTEXT('','3D')
);
#38507=(
GEOMETRIC_REPRESENTATION_CONTEXT(3)
GLOBAL_UNCERTAINTY_ASSIGNED_CONTEXT((#38490))
GLOBAL_UNIT_ASSIGNED_CONTEXT((#38508,#38510,#38511))
REPRESENTATION_CONTEXT('','3D')
);
#38508=(
LENGTH_UNIT()
NAMED_UNIT(*)
SI_UNIT(.MILLI.,.METRE.)
);
#38510=(
NAMED_UNIT(*)
PLANE_ANGLE_UNIT()
SI_UNIT($,.RADIAN.)
);
#38511=(
NAMED_UNIT(*)
SI_UNIT($,.STERADIAN.)
SOLID_ANGLE_UNIT()
);
#38525=SHAPE_DEFINITION_REPRESENTATION(#38541,#38587);
#38541=PRODUCT_DEFINITION_SHAPE('',$,#38604);
#38587=SHAPE_REPRESENTATION('',(#16304),#38504);
#38590=PRODUCT_DEFINITION_CONTEXT('part definition',#38640,'design');
#38604=PRODUCT_DEFINITION('2026-10-26-01-10-50-044',
'07_Slipper_Retainer_Plate',#38620,#38590);
#38620=PRODUCT_DEFINITION_FORMATION('',$,#38655);
#38640=APPLICATION_CONTEXT(
'Core Data for Automotive Mechanical Design Process');
#38641=PRODUCT_CONTEXT('part definition',#38640,'mechanical');
#38655=PRODUCT('2026-10-26-01-10-50-044','07_Slipper_Retainer_Plate',$,
(#38641));
#38707=COLOUR_RGB('Sky Blue',0.24,0.69,0.87);
#38708=FILL_AREA_STYLE_COLOUR('',#38707);
#38709=FILL_AREA_STYLE('',(#38708));
#38710=SURFACE_STYLE_FILL_AREA(#38709);
#38711=SURFACE_SIDE_STYLE('',(#38710));
#38712=SURFACE_STYLE_USAGE(.BOTH.,#38711);
#38713=PRESENTATION_STYLE_ASSIGNMENT((#38712));
ENDSEC;
END-ISO-10303-21;
